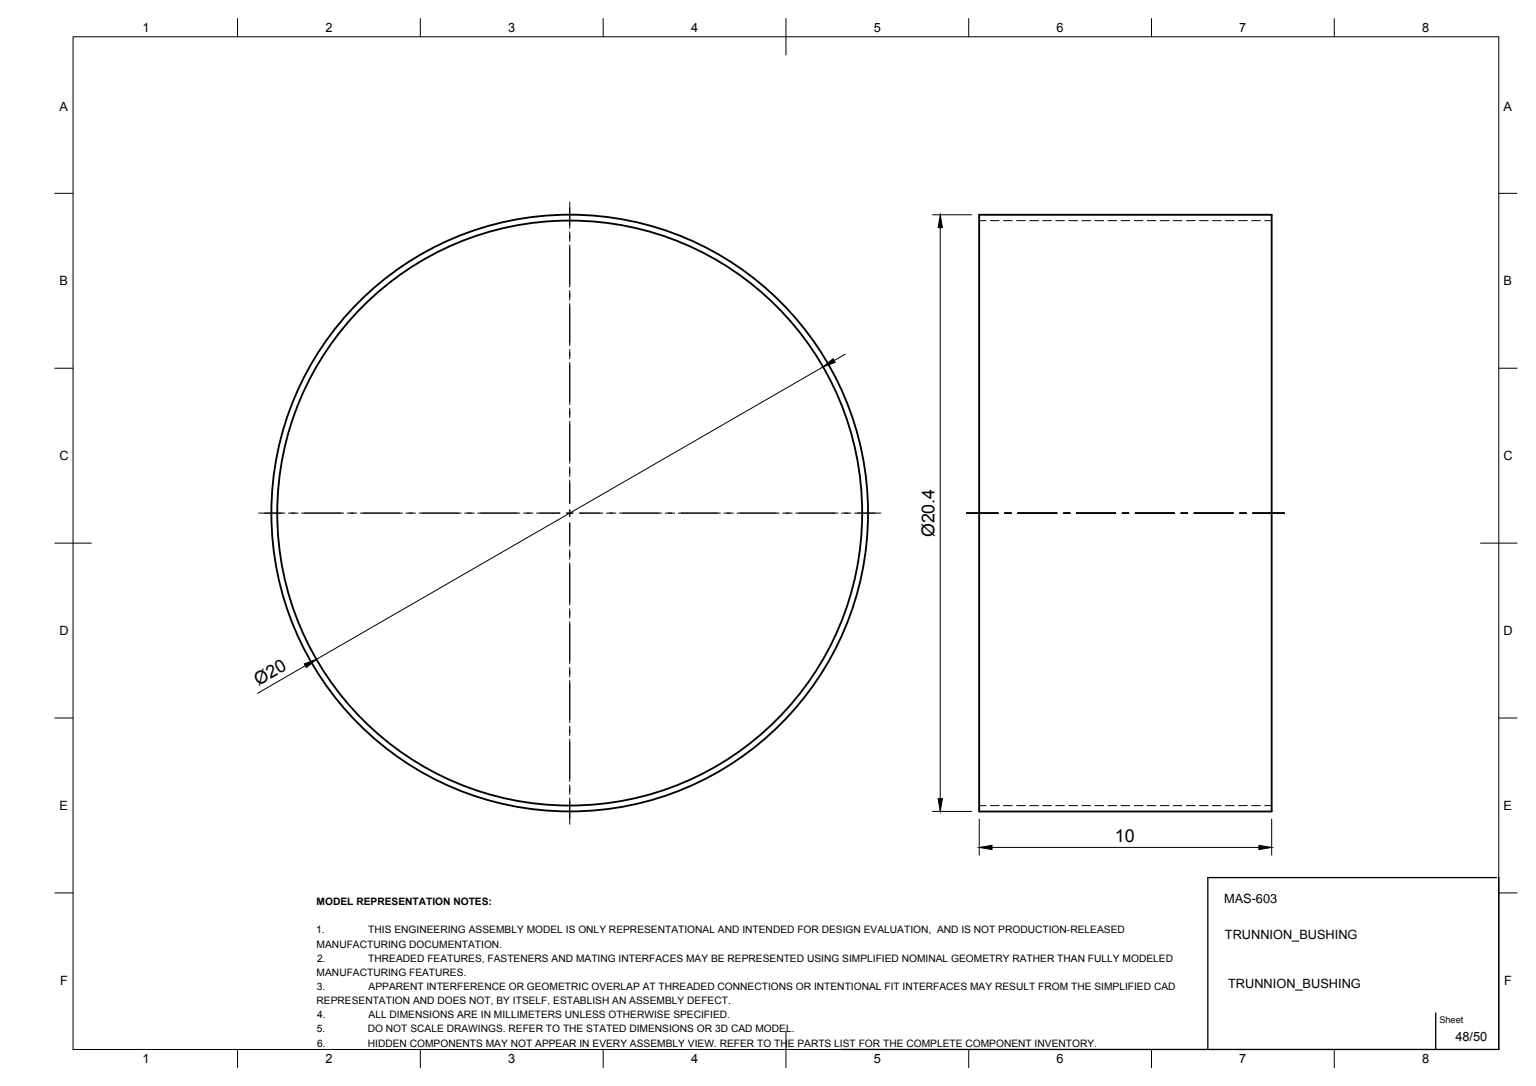
ISO-10303-21;
HEADER;
FILE_DESCRIPTION((''),'2;1');
FILE_NAME('TRUNNION_BUSHING.step','2026-10-01T22:06:14-07:00',(''),(''),'','','');
FILE_SCHEMA (('AUTOMOTIVE_DESIGN { 1 0 10303 214 3 1 1 }'));
ENDSEC;
DATA;
#10=MECHANICAL_DESIGN_GEOMETRIC_PRESENTATION_REPRESENTATION('',(#1026),#50440);
#926=SHAPE_REPRESENTATION_RELATIONSHIP('SRR','None',#50660,#971) ;
#971=ADVANCED_BREP_SHAPE_REPRESENTATION('',(#1079),#50429) ;
#1026=STYLED_ITEM('',(#50887),#1079) ;
#1079=MANIFOLD_SOLID_BREP('TRUNNION_BUSHING',#28704) ;
#1396=FACE_BOUND('',#5632,.T.) ;
#1397=FACE_BOUND('',#5634,.T.) ;
#2274=PLANE('',#32164) ;
#2275=PLANE('',#32165) ;
#3791=FACE_OUTER_BOUND('',#5629,.T.) ;
#3792=FACE_OUTER_BOUND('',#5630,.T.) ;
#3793=FACE_OUTER_BOUND('',#5631,.T.) ;
#3794=FACE_OUTER_BOUND('',#5633,.T.) ;
#5629=EDGE_LOOP('',(#26187,#26188,#26189,#26190)) ;
#5630=EDGE_LOOP('',(#26191,#26192,#26193,#26194)) ;
#5631=EDGE_LOOP('',(#26195)) ;
#5632=EDGE_LOOP('',(#26196)) ;
#5633=EDGE_LOOP('',(#26197)) ;
#5634=EDGE_LOOP('',(#26198)) ;
#8075=LINE('',#49766,#10547) ;
#8076=LINE('',#49772,#10548) ;
#10547=VECTOR('',#40620,1.) ;
#10548=VECTOR('',#40627,1.02) ;
#11791=CIRCLE('',#32159,1.) ;
#11792=CIRCLE('',#32160,1.) ;
#11793=CIRCLE('',#32162,1.02) ;
#11794=CIRCLE('',#32163,1.02) ;
#14408=VERTEX_POINT('',#49763) ;
#14409=VERTEX_POINT('',#49765) ;
#14410=VERTEX_POINT('',#49769) ;
#14411=VERTEX_POINT('',#49771) ;
#18359=EDGE_CURVE('',#14408,#14408,#11791,.T.) ;
#18360=EDGE_CURVE('',#14408,#14409,#8075,.T.) ;
#18361=EDGE_CURVE('',#14409,#14409,#11792,.T.) ;
#18362=EDGE_CURVE('',#14410,#14410,#11793,.T.) ;
#18363=EDGE_CURVE('',#14410,#14411,#8076,.T.) ;
#18364=EDGE_CURVE('',#14411,#14411,#11794,.T.) ;
#26187=ORIENTED_EDGE('',*,*,#18359,.F.) ;
#26188=ORIENTED_EDGE('',*,*,#18360,.T.) ;
#26189=ORIENTED_EDGE('',*,*,#18361,.F.) ;
#26190=ORIENTED_EDGE('',*,*,#18360,.F.) ;
#26191=ORIENTED_EDGE('',*,*,#18362,.F.) ;
#26192=ORIENTED_EDGE('',*,*,#18363,.T.) ;
#26193=ORIENTED_EDGE('',*,*,#18364,.F.) ;
#26194=ORIENTED_EDGE('',*,*,#18363,.F.) ;
#26195=ORIENTED_EDGE('',*,*,#18364,.T.) ;
#26196=ORIENTED_EDGE('',*,*,#18359,.T.) ;
#26197=ORIENTED_EDGE('',*,*,#18362,.T.) ;
#26198=ORIENTED_EDGE('',*,*,#18361,.T.) ;
#27049=CYLINDRICAL_SURFACE('',#32158,1.) ;
#27050=CYLINDRICAL_SURFACE('',#32161,1.02) ;
#28526=ADVANCED_FACE('',(#3791),#27049,.F.) ;
#28527=ADVANCED_FACE('',(#3792),#27050,.T.) ;
#28528=ADVANCED_FACE('',(#3793,#1396),#2274,.T.) ;
#28529=ADVANCED_FACE('',(#3794,#1397),#2275,.T.) ;
#28704=CLOSED_SHELL('',(#28526,#28527,#28528,#28529)) ;
#32157=AXIS2_PLACEMENT_3D('',#49761,#40614,#40615) ;
#32158=AXIS2_PLACEMENT_3D('',#49762,#40616,#40617) ;
#32159=AXIS2_PLACEMENT_3D('',#49764,#40618,#40619) ;
#32160=AXIS2_PLACEMENT_3D('',#49767,#40621,#40622) ;
#32161=AXIS2_PLACEMENT_3D('',#49768,#40623,#40624) ;
#32162=AXIS2_PLACEMENT_3D('',#49770,#40625,#40626) ;
#32163=AXIS2_PLACEMENT_3D('',#49773,#40628,#40629) ;
#32164=AXIS2_PLACEMENT_3D('',#49774,#40630,#40631) ;
#32165=AXIS2_PLACEMENT_3D('',#49775,#40632,#40633) ;
#40614=DIRECTION('axis',(0.,0.,1.)) ;
#40615=DIRECTION('refdir',(1.,0.,0.)) ;
#40616=DIRECTION('center_axis',(1.,0.,0.)) ;
#40617=DIRECTION('ref_axis',(0.,0.,-1.)) ;
#40618=DIRECTION('center_axis',(1.,0.,0.)) ;
#40619=DIRECTION('ref_axis',(0.,0.,-1.)) ;
#40620=DIRECTION('',(1.,0.,0.)) ;
#40621=DIRECTION('center_axis',(-1.,0.,0.)) ;
#40622=DIRECTION('ref_axis',(0.,0.,-1.)) ;
#40623=DIRECTION('center_axis',(1.,0.,0.)) ;
#40624=DIRECTION('ref_axis',(0.,0.,-1.)) ;
#40625=DIRECTION('center_axis',(1.,0.,0.)) ;
#40626=DIRECTION('ref_axis',(0.,0.,-1.)) ;
#40627=DIRECTION('',(-1.,0.,0.)) ;
#40628=DIRECTION('center_axis',(-1.,0.,0.)) ;
#40629=DIRECTION('ref_axis',(0.,0.,-1.)) ;
#40630=DIRECTION('center_axis',(-1.,0.,0.)) ;
#40631=DIRECTION('ref_axis',(0.,0.,1.)) ;
#40632=DIRECTION('center_axis',(1.,0.,0.)) ;
#40633=DIRECTION('ref_axis',(0.,0.,-1.)) ;
#49761=CARTESIAN_POINT('',(0.,0.,0.)) ;
#49762=CARTESIAN_POINT('Origin',(10.,0.,24.)) ;
#49763=CARTESIAN_POINT('',(9.5,-1.22464679914735E-16,25.)) ;
#49764=CARTESIAN_POINT('Origin',(9.5,0.,24.)) ;
#49765=CARTESIAN_POINT('',(10.5,1.22464679914735E-16,25.)) ;
#49766=CARTESIAN_POINT('',(10.,-1.22464679914735E-16,25.)) ;
#49767=CARTESIAN_POINT('Origin',(10.5,0.,24.)) ;
#49768=CARTESIAN_POINT('Origin',(10.,0.,24.)) ;
#49769=CARTESIAN_POINT('',(10.5,-1.2491397351303E-16,25.02)) ;
#49770=CARTESIAN_POINT('Origin',(10.5,0.,24.)) ;
#49771=CARTESIAN_POINT('',(9.5,-1.2491397351303E-16,25.02)) ;
#49772=CARTESIAN_POINT('',(10.,-1.2491397351303E-16,25.02)) ;
#49773=CARTESIAN_POINT('Origin',(9.5,0.,24.)) ;
#49774=CARTESIAN_POINT('Origin',(9.5,0.,24.)) ;
#49775=CARTESIAN_POINT('Origin',(10.5,0.,24.)) ;
#50376=UNCERTAINTY_MEASURE_WITH_UNIT(LENGTH_MEASURE(0.001),#50441,
'DISTANCE_ACCURACY_VALUE',
'Maximum model space distance between geometric entities at asserted c
onnectivities') ;
#50387=UNCERTAINTY_MEASURE_WITH_UNIT(LENGTH_MEASURE(0.001),#50441,
'DISTANCE_ACCURACY_VALUE',
'Maximum model space distance between geometric entities at asserted c
onnectivities') ;
#50429=(
GEOMETRIC_REPRESENTATION_CONTEXT(3)
GLOBAL_UNCERTAINTY_ASSIGNED_CONTEXT((#50376))
GLOBAL_UNIT_ASSIGNED_CONTEXT((#50441,#50443,#50444))
REPRESENTATION_CONTEXT('','3D')
) ;
#50440=(
GEOMETRIC_REPRESENTATION_CONTEXT(3)
GLOBAL_UNCERTAINTY_ASSIGNED_CONTEXT((#50387))
GLOBAL_UNIT_ASSIGNED_CONTEXT((#50441,#50443,#50444))
REPRESENTATION_CONTEXT('','3D')
) ;
#50441=(
LENGTH_UNIT()
NAMED_UNIT(*)
SI_UNIT(.CENTI.,.METRE.)
) ;
#50443=(
NAMED_UNIT(*)
PLANE_ANGLE_UNIT()
SI_UNIT($,.RADIAN.)
) ;
#50444=(
NAMED_UNIT(*)
SI_UNIT($,.STERADIAN.)
SOLID_ANGLE_UNIT()
) ;
#50486=SHAPE_DEFINITION_REPRESENTATION(#50576,#50660) ;
#50576=PRODUCT_DEFINITION_SHAPE('',$,#50713) ;
#50660=SHAPE_REPRESENTATION('',(#32157),#50429) ;
#50671=PRODUCT_DEFINITION_CONTEXT('part definition',#50829,'design') ;
#50713=PRODUCT_DEFINITION('TRUNNION_BUSHING','TRUNNION_BUSHING',
#50765,#50671) ;
#50765=PRODUCT_DEFINITION_FORMATION('',$,#50872) ;
#50829=APPLICATION_CONTEXT(
'Core Data for Automotive Mechanical Design Process') ;
#50830=PRODUCT_CONTEXT('part definition',#50829,'mechanical') ;
#50872=PRODUCT('TRUNNION_BUSHING','TRUNNION_BUSHING',$,(#50830)) ;
#50887=PRESENTATION_STYLE_ASSIGNMENT((#50894)) ;
#50894=SURFACE_STYLE_USAGE(.BOTH.,#50901) ;
#50901=SURFACE_SIDE_STYLE('',(#50908)) ;
#50908=SURFACE_STYLE_FILL_AREA(#50915) ;
#50915=FILL_AREA_STYLE('Brass - Polished',(#50922)) ;
#50922=FILL_AREA_STYLE_COLOUR('Brass - Polished',#50929) ;
#50929=COLOUR_RGB('Brass - Polished', 0.66274510, 0.83137255, 0.94901961) ;
ENDSEC;
END-ISO-10303-21;
